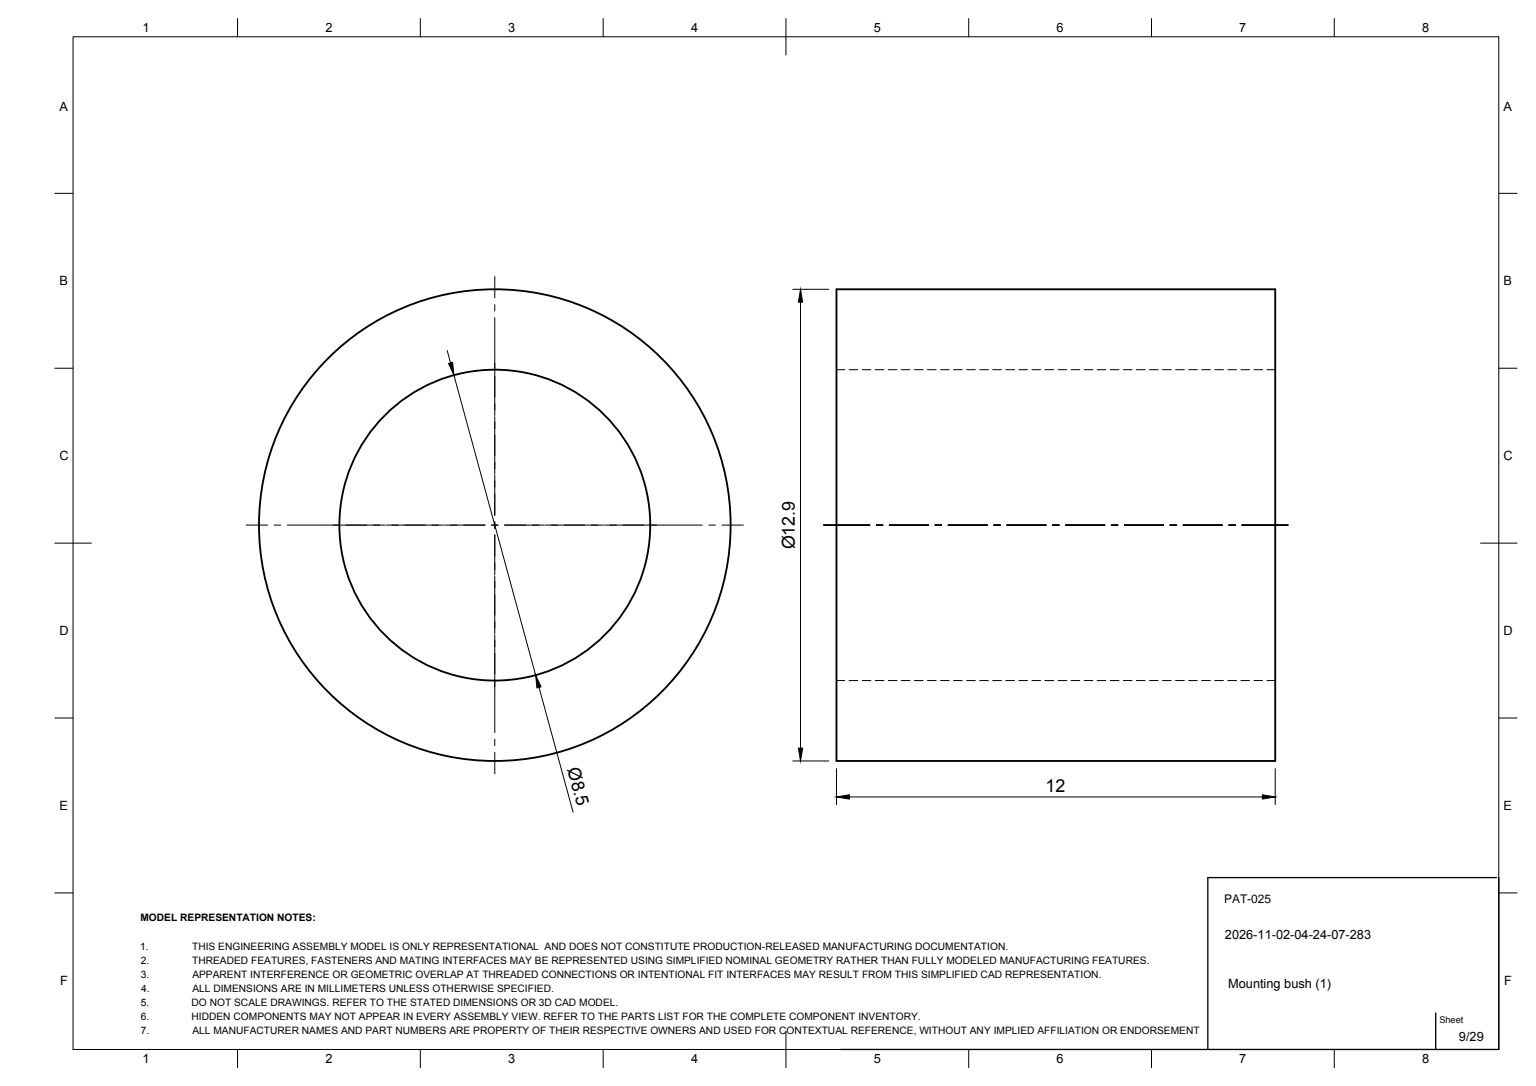
ISO-10303-21;
HEADER;
/* Generated by software containing ST-Developer
 * from STEP Tools, Inc. (www.steptools.com) 
 */

FILE_DESCRIPTION(
/* description */ ('Counter shaft with two pulleys and keyed hub'),
/* implementation_level */ '2;1');

FILE_NAME(
/* name */ 'Mounting bush (1).step',
/* time_stamp */ '2026-10-27T10:46:10-07:00',
/* author */ (''),
/* organization */ (''),
/* preprocessor_version */ 'ST-DEVELOPER v20.2',
/* originating_system */ 'Autodesk Translation Framework v15.17.0.0',
/* authorisation */ '');

FILE_SCHEMA (('AUTOMOTIVE_DESIGN { 1 0 10303 214 3 1 1 }'));
ENDSEC;

DATA;
#10=MECHANICAL_DESIGN_GEOMETRIC_PRESENTATION_REPRESENTATION('',(#294),#10821);
#244=SHAPE_REPRESENTATION_RELATIONSHIP('SRR','None',#10930,#269);
#269=ADVANCED_BREP_SHAPE_REPRESENTATION('',(#320),#10798);
#294=STYLED_ITEM('',(#11128),#320);
#320=MANIFOLD_SOLID_BREP('Body1',#5577);
#350=FACE_BOUND('',#941,.T.);
#351=FACE_BOUND('',#943,.T.);
#451=PLANE('',#5928);
#452=PLANE('',#5929);
#614=FACE_OUTER_BOUND('',#938,.T.);
#615=FACE_OUTER_BOUND('',#939,.T.);
#616=FACE_OUTER_BOUND('',#940,.T.);
#617=FACE_OUTER_BOUND('',#942,.T.);
#938=EDGE_LOOP('',(#3737,#3738,#3739,#3740));
#939=EDGE_LOOP('',(#3741,#3742,#3743,#3744));
#940=EDGE_LOOP('',(#3745));
#941=EDGE_LOOP('',(#3746));
#942=EDGE_LOOP('',(#3747));
#943=EDGE_LOOP('',(#3748));
#1349=LINE('',#8439,#1738);
#1350=LINE('',#8445,#1739);
#1738=VECTOR('',#6695,0.425);
#1739=VECTOR('',#6702,0.645);
#2097=CIRCLE('',#5923,0.425);
#2098=CIRCLE('',#5924,0.425);
#2099=CIRCLE('',#5926,0.645);
#2100=CIRCLE('',#5927,0.645);
#2420=VERTEX_POINT('',#8436);
#2421=VERTEX_POINT('',#8438);
#2422=VERTEX_POINT('',#8442);
#2423=VERTEX_POINT('',#8444);
#2941=EDGE_CURVE('',#2420,#2420,#2097,.T.);
#2942=EDGE_CURVE('',#2420,#2421,#1349,.T.);
#2943=EDGE_CURVE('',#2421,#2421,#2098,.T.);
#2944=EDGE_CURVE('',#2422,#2422,#2099,.T.);
#2945=EDGE_CURVE('',#2422,#2423,#1350,.T.);
#2946=EDGE_CURVE('',#2423,#2423,#2100,.T.);
#3737=ORIENTED_EDGE('',*,*,#2941,.F.);
#3738=ORIENTED_EDGE('',*,*,#2942,.T.);
#3739=ORIENTED_EDGE('',*,*,#2943,.T.);
#3740=ORIENTED_EDGE('',*,*,#2942,.F.);
#3741=ORIENTED_EDGE('',*,*,#2944,.F.);
#3742=ORIENTED_EDGE('',*,*,#2945,.T.);
#3743=ORIENTED_EDGE('',*,*,#2946,.T.);
#3744=ORIENTED_EDGE('',*,*,#2945,.F.);
#3745=ORIENTED_EDGE('',*,*,#2944,.T.);
#3746=ORIENTED_EDGE('',*,*,#2941,.T.);
#3747=ORIENTED_EDGE('',*,*,#2946,.F.);
#3748=ORIENTED_EDGE('',*,*,#2943,.F.);
#5119=CYLINDRICAL_SURFACE('',#5922,0.425);
#5120=CYLINDRICAL_SURFACE('',#5925,0.645);
#5285=ADVANCED_FACE('',(#614),#5119,.F.);
#5286=ADVANCED_FACE('',(#615),#5120,.T.);
#5287=ADVANCED_FACE('',(#616,#350),#451,.T.);
#5288=ADVANCED_FACE('',(#617,#351),#452,.F.);
#5577=CLOSED_SHELL('',(#5285,#5286,#5287,#5288));
#5921=AXIS2_PLACEMENT_3D('',#8434,#6689,#6690);
#5922=AXIS2_PLACEMENT_3D('',#8435,#6691,#6692);
#5923=AXIS2_PLACEMENT_3D('',#8437,#6693,#6694);
#5924=AXIS2_PLACEMENT_3D('',#8440,#6696,#6697);
#5925=AXIS2_PLACEMENT_3D('',#8441,#6698,#6699);
#5926=AXIS2_PLACEMENT_3D('',#8443,#6700,#6701);
#5927=AXIS2_PLACEMENT_3D('',#8446,#6703,#6704);
#5928=AXIS2_PLACEMENT_3D('',#8447,#6705,#6706);
#5929=AXIS2_PLACEMENT_3D('',#8448,#6707,#6708);
#6689=DIRECTION('axis',(0.,0.,1.));
#6690=DIRECTION('refdir',(1.,0.,0.));
#6691=DIRECTION('center_axis',(0.,0.,1.));
#6692=DIRECTION('ref_axis',(1.,0.,0.));
#6693=DIRECTION('center_axis',(0.,0.,-1.));
#6694=DIRECTION('ref_axis',(1.,0.,0.));
#6695=DIRECTION('',(0.,0.,-1.));
#6696=DIRECTION('center_axis',(0.,0.,-1.));
#6697=DIRECTION('ref_axis',(1.,0.,0.));
#6698=DIRECTION('center_axis',(0.,0.,1.));
#6699=DIRECTION('ref_axis',(1.,0.,0.));
#6700=DIRECTION('center_axis',(0.,0.,1.));
#6701=DIRECTION('ref_axis',(1.,0.,0.));
#6702=DIRECTION('',(0.,0.,-1.));
#6703=DIRECTION('center_axis',(0.,0.,1.));
#6704=DIRECTION('ref_axis',(1.,0.,0.));
#6705=DIRECTION('center_axis',(0.,0.,1.));
#6706=DIRECTION('ref_axis',(1.,0.,0.));
#6707=DIRECTION('center_axis',(0.,0.,1.));
#6708=DIRECTION('ref_axis',(1.,0.,0.));
#8434=CARTESIAN_POINT('',(0.,0.,0.));
#8435=CARTESIAN_POINT('Origin',(4.75,0.,1.2));
#8436=CARTESIAN_POINT('',(4.325,-5.20474889637625E-17,2.4));
#8437=CARTESIAN_POINT('Origin',(4.75,0.,2.4));
#8438=CARTESIAN_POINT('',(4.325,-5.20474889637625E-17,1.2));
#8439=CARTESIAN_POINT('',(4.325,-5.20474889637625E-17,1.2));
#8440=CARTESIAN_POINT('Origin',(4.75,0.,1.2));
#8441=CARTESIAN_POINT('Origin',(4.75,0.,1.2));
#8442=CARTESIAN_POINT('',(4.105,-7.89897185450042E-17,2.4));
#8443=CARTESIAN_POINT('Origin',(4.75,0.,2.4));
#8444=CARTESIAN_POINT('',(4.105,-7.89897185450042E-17,1.2));
#8445=CARTESIAN_POINT('',(4.105,-7.89897185450042E-17,1.2));
#8446=CARTESIAN_POINT('Origin',(4.75,0.,1.2));
#8447=CARTESIAN_POINT('Origin',(4.75,0.,2.4));
#8448=CARTESIAN_POINT('Origin',(4.75,0.,1.2));
#10768=UNCERTAINTY_MEASURE_WITH_UNIT(LENGTH_MEASURE(0.001),#10822,
'DISTANCE_ACCURACY_VALUE',
'Maximum model space distance between geometric entities at asserted c
onnectivities');
#10791=UNCERTAINTY_MEASURE_WITH_UNIT(LENGTH_MEASURE(0.001),#10822,
'DISTANCE_ACCURACY_VALUE',
'Maximum model space distance between geometric entities at asserted c
onnectivities');
#10798=(
GEOMETRIC_REPRESENTATION_CONTEXT(3)
GLOBAL_UNCERTAINTY_ASSIGNED_CONTEXT((#10768))
GLOBAL_UNIT_ASSIGNED_CONTEXT((#10822,#10824,#10825))
REPRESENTATION_CONTEXT('','3D')
);
#10821=(
GEOMETRIC_REPRESENTATION_CONTEXT(3)
GLOBAL_UNCERTAINTY_ASSIGNED_CONTEXT((#10791))
GLOBAL_UNIT_ASSIGNED_CONTEXT((#10822,#10824,#10825))
REPRESENTATION_CONTEXT('','3D')
);
#10822=(
LENGTH_UNIT()
NAMED_UNIT(*)
SI_UNIT(.CENTI.,.METRE.)
);
#10824=(
NAMED_UNIT(*)
PLANE_ANGLE_UNIT()
SI_UNIT($,.RADIAN.)
);
#10825=(
NAMED_UNIT(*)
SI_UNIT($,.STERADIAN.)
SOLID_ANGLE_UNIT()
);
#10832=SHAPE_DEFINITION_REPRESENTATION(#10861,#10930);
#10861=PRODUCT_DEFINITION_SHAPE('',$,#10960);
#10930=SHAPE_REPRESENTATION('',(#5921),#10798);
#10953=PRODUCT_DEFINITION_CONTEXT('part definition',#11042,'design');
#10960=PRODUCT_DEFINITION('Mounting bush (1)','Mounting bush (1)',#10989,
#10953);
#10989=PRODUCT_DEFINITION_FORMATION('',$,#11050);
#11042=APPLICATION_CONTEXT(
'Core Data for Automotive Mechanical Design Process');
#11043=PRODUCT_CONTEXT('part definition',#11042,'mechanical');
#11050=PRODUCT('Mounting bush (1)','Mounting bush (1)','Mounting bush (1)',(#11043));
#11122=COLOUR_RGB('Sky Blue',0.24,0.69,0.87);
#11123=FILL_AREA_STYLE_COLOUR('',#11122);
#11124=FILL_AREA_STYLE('',(#11123));
#11125=SURFACE_STYLE_FILL_AREA(#11124);
#11126=SURFACE_SIDE_STYLE('',(#11125));
#11127=SURFACE_STYLE_USAGE(.BOTH.,#11126);
#11128=PRESENTATION_STYLE_ASSIGNMENT((#11127));
ENDSEC;
END-ISO-10303-21;
